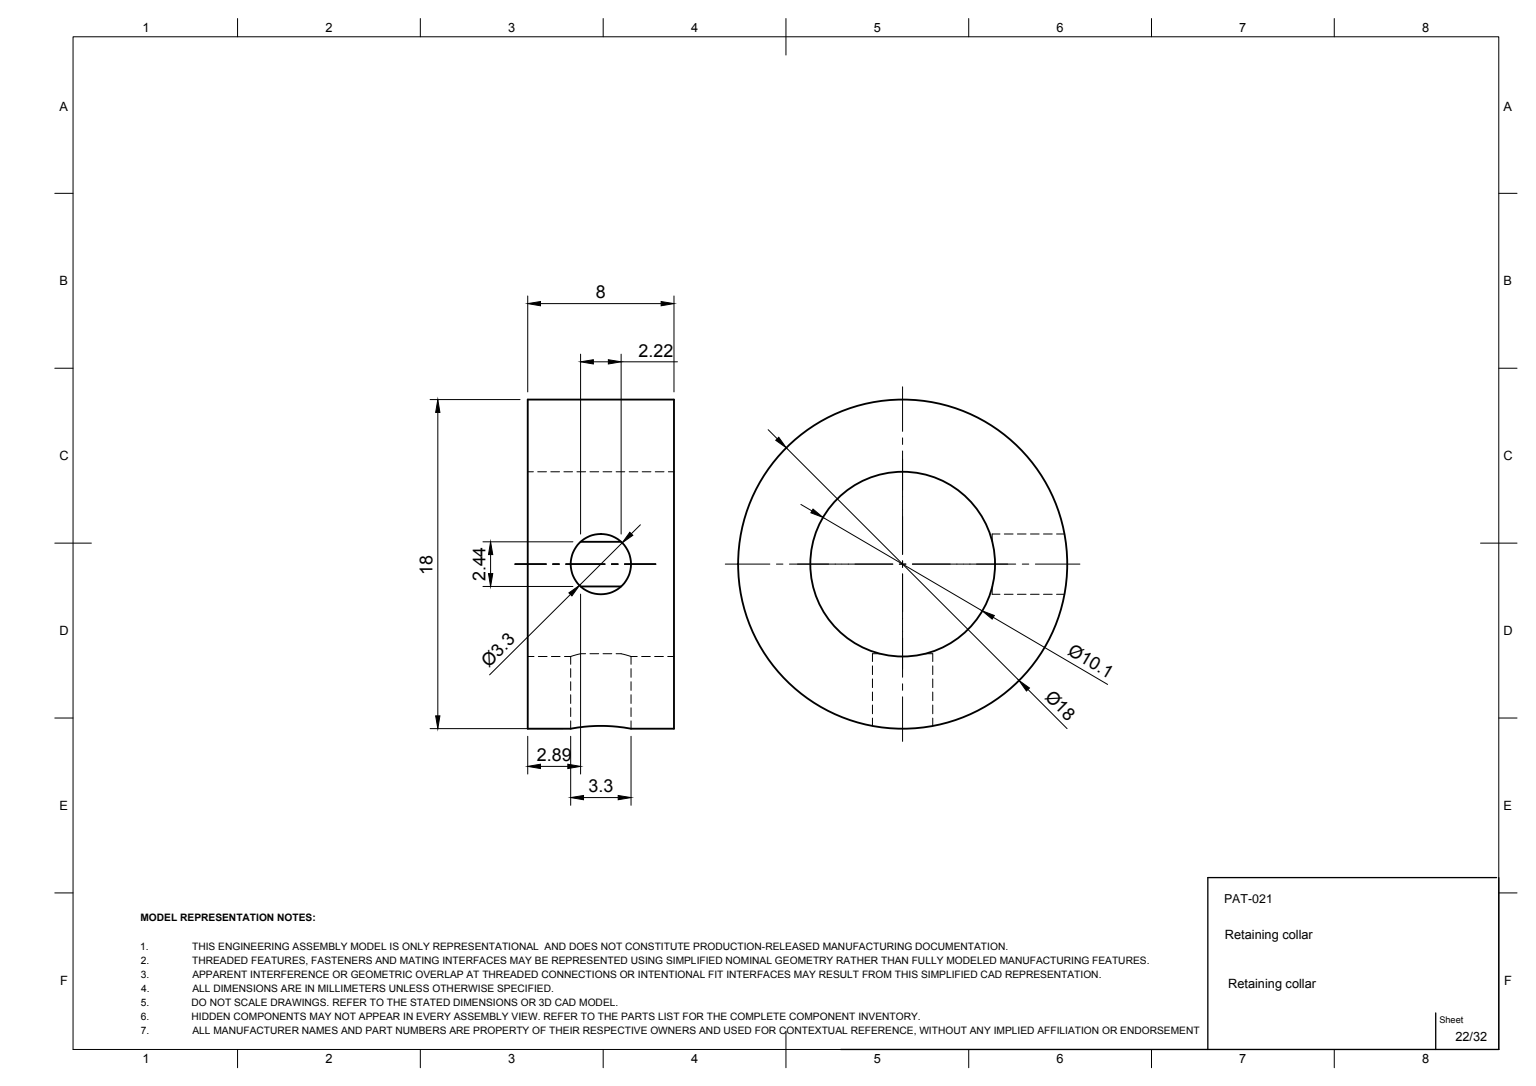
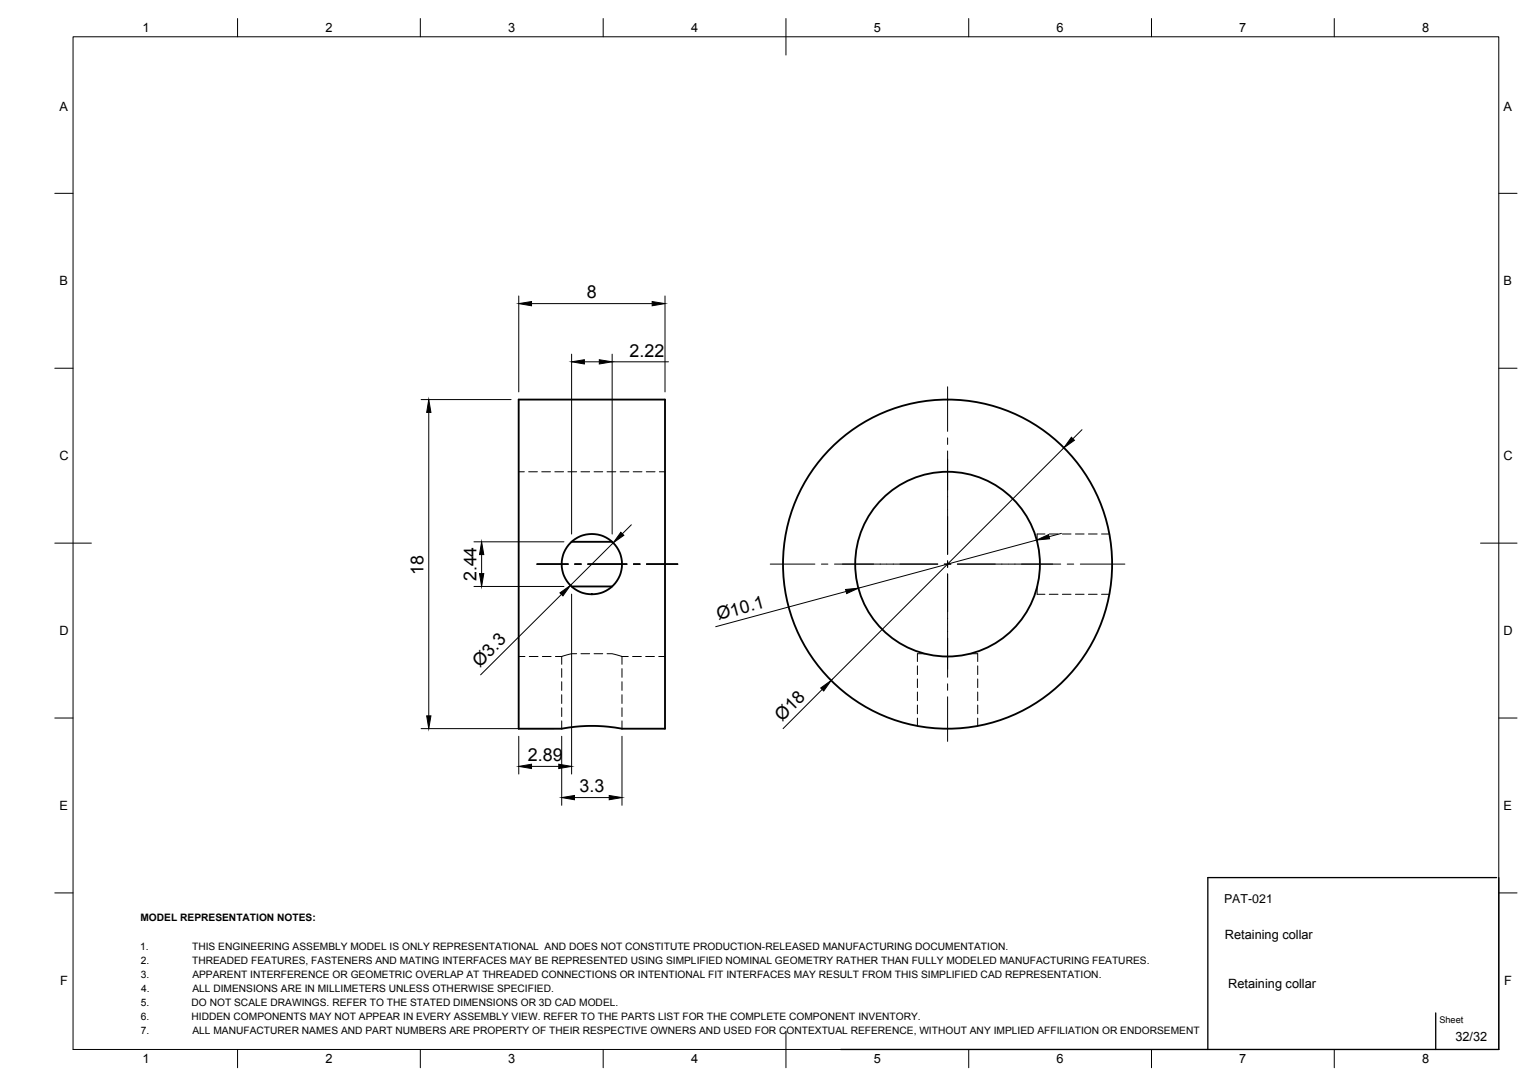
ISO-10303-21;
HEADER;
/* Generated by software containing ST-Developer
 * from STEP Tools, Inc. (www.steptools.com) 
 */

FILE_DESCRIPTION(
/* description */ ('Chain-less indexing wheel (Geneva) drive'),
/* implementation_level */ '2;1');

FILE_NAME(
/* name */ 'Retaining collar.step',
/* time_stamp */ '2026-10-28T03:25:22-07:00',
/* author */ (''),
/* organization */ (''),
/* preprocessor_version */ 'ST-DEVELOPER v20.2',
/* originating_system */ 'Autodesk Translation Framework v15.17.0.0',
/* authorisation */ '');

FILE_SCHEMA (('AUTOMOTIVE_DESIGN { 1 0 10303 214 3 1 1 }'));
ENDSEC;

DATA;
#10=MECHANICAL_DESIGN_GEOMETRIC_PRESENTATION_REPRESENTATION('',(#325),#10957);
#233=B_SPLINE_CURVE_WITH_KNOTS('',3,(#9946,#9947,#9948,#9949,#9950,#9951,
#9952,#9953,#9954,#9955,#9956,#9957,#9958,#9959,#9960,#9961,#9962,#9963,
#9964,#9965,#9966,#9967,#9968,#9969,#9970,#9971,#9972,#9973,#9974,#9975,
#9976,#9977,#9978,#9979),.UNSPECIFIED.,.T.,.F.,(4,2,2,2,2,2,2,2,2,2,2,2,
2,2,2,2,4),(0.,0.0623062782223143,0.124612556444629,0.186916384615149,0.249220212785669,
0.31152404095619,0.37382786912671,0.436134147349024,0.498440425571339,0.560746703793653,
0.623052982015967,0.685356810186488,0.747660638357008,0.809964466527529,
0.872268294698049,0.934574572920363,0.996880851142677),.UNSPECIFIED.);
#234=B_SPLINE_CURVE_WITH_KNOTS('',3,(#9982,#9983,#9984,#9985,#9986,#9987,
#9988,#9989,#9990,#9991,#9992,#9993,#9994,#9995),.UNSPECIFIED.,.F.,.F.,
(4,2,2,2,2,2,4),(0.618551524396292,0.626563103102765,0.689203386094988,
0.751843669087211,0.814483952079434,0.877124235071657,0.88513581377813),
 .UNSPECIFIED.);
#235=B_SPLINE_CURVE_WITH_KNOTS('',3,(#9998,#9999,#10000,#10001,#10002,#10003,
#10004,#10005,#10006,#10007,#10008,#10009,#10010,#10011),.UNSPECIFIED.,
 .F.,.F.,(4,2,2,2,2,2,4),(0.117322411671485,0.125333990377958,0.187974273370181,
0.250614556362404,0.313254839354627,0.37589512234685,0.383906701053323),
 .UNSPECIFIED.);
#236=B_SPLINE_CURVE_WITH_KNOTS('',3,(#10022,#10023,#10024,#10025,#10026,
#10027,#10028,#10029,#10030,#10031),.UNSPECIFIED.,.F.,.F.,(4,2,2,2,4),(0.,
0.0623062782223142,0.124612556444628,0.186916384615149,0.249220212785669),
 .UNSPECIFIED.);
#237=B_SPLINE_CURVE_WITH_KNOTS('',3,(#10033,#10034,#10035,#10036,#10037,
#10038,#10039,#10040,#10041,#10042),.UNSPECIFIED.,.F.,.F.,(4,2,2,2,4),(0.747660638357008,
0.809964466527529,0.872268294698049,0.934574572920363,0.996880851142677),
 .UNSPECIFIED.);
#238=B_SPLINE_CURVE_WITH_KNOTS('',3,(#10043,#10044,#10045,#10046,#10047,
#10048,#10049,#10050,#10051,#10052,#10053,#10054,#10055,#10056,#10057,#10058,
#10059,#10060),.UNSPECIFIED.,.F.,.F.,(4,2,2,2,2,2,2,2,4),(0.249220212785669,
0.31152404095619,0.37382786912671,0.436134147349024,0.498440425571339,0.560746703793653,
0.623052982015967,0.685356810186488,0.747660638357008),.UNSPECIFIED.);
#239=B_SPLINE_CURVE_WITH_KNOTS('',3,(#10064,#10065,#10066,#10067,#10068,
#10069,#10070,#10071),.UNSPECIFIED.,.F.,.F.,(4,2,2,4),(0.618551524396292,
0.626563103102765,0.689203386094988,0.751843669087211),.UNSPECIFIED.);
#240=B_SPLINE_CURVE_WITH_KNOTS('',3,(#10075,#10076,#10077,#10078,#10079,
#10080,#10081,#10082),.UNSPECIFIED.,.F.,.F.,(4,2,2,4),(0.250614556362404,
0.313254839354627,0.37589512234685,0.383906701053323),.UNSPECIFIED.);
#241=B_SPLINE_CURVE_WITH_KNOTS('',3,(#10083,#10084,#10085,#10086,#10087,
#10088,#10089,#10090),.UNSPECIFIED.,.F.,.F.,(4,2,2,4),(0.117322411671484,
0.125333990377958,0.187974273370181,0.250614556362404),.UNSPECIFIED.);
#242=B_SPLINE_CURVE_WITH_KNOTS('',3,(#10091,#10092,#10093,#10094,#10095,
#10096,#10097,#10098),.UNSPECIFIED.,.F.,.F.,(4,2,2,4),(0.751843669087211,
0.814483952079434,0.877124235071657,0.885135813778131),.UNSPECIFIED.);
#267=SHAPE_REPRESENTATION_RELATIONSHIP('SRR','None',#11082,#292);
#292=ADVANCED_BREP_SHAPE_REPRESENTATION('',(#357),#10945);
#325=STYLED_ITEM('',(#11301),#357);
#357=MANIFOLD_SOLID_BREP('Body1',#5722);
#441=FACE_BOUND('',#1265,.T.);
#442=FACE_BOUND('',#1267,.T.);
#443=FACE_BOUND('',#1269,.T.);
#444=FACE_BOUND('',#1271,.T.);
#569=PLANE('',#6451);
#570=PLANE('',#6456);
#571=PLANE('',#6457);
#572=PLANE('',#6461);
#573=PLANE('',#6468);
#574=PLANE('',#6469);
#851=FACE_OUTER_BOUND('',#1258,.T.);
#852=FACE_OUTER_BOUND('',#1259,.T.);
#853=FACE_OUTER_BOUND('',#1260,.T.);
#854=FACE_OUTER_BOUND('',#1261,.T.);
#855=FACE_OUTER_BOUND('',#1262,.T.);
#856=FACE_OUTER_BOUND('',#1263,.T.);
#857=FACE_OUTER_BOUND('',#1264,.T.);
#858=FACE_OUTER_BOUND('',#1266,.T.);
#859=FACE_OUTER_BOUND('',#1268,.T.);
#860=FACE_OUTER_BOUND('',#1270,.T.);
#1258=EDGE_LOOP('',(#4601,#4602,#4603));
#1259=EDGE_LOOP('',(#4604,#4605,#4606,#4607,#4608,#4609,#4610,#4611));
#1260=EDGE_LOOP('',(#4612,#4613));
#1261=EDGE_LOOP('',(#4614,#4615));
#1262=EDGE_LOOP('',(#4616,#4617,#4618,#4619,#4620,#4621,#4622,#4623,#4624,
#4625,#4626));
#1263=EDGE_LOOP('',(#4627,#4628));
#1264=EDGE_LOOP('',(#4629,#4630,#4631,#4632,#4633,#4634,#4635,#4636,#4637,
#4638,#4639,#4640));
#1265=EDGE_LOOP('',(#4641,#4642,#4643,#4644));
#1266=EDGE_LOOP('',(#4645,#4646,#4647,#4648,#4649,#4650,#4651,#4652,#4653));
#1267=EDGE_LOOP('',(#4654));
#1268=EDGE_LOOP('',(#4655));
#1269=EDGE_LOOP('',(#4656));
#1270=EDGE_LOOP('',(#4657));
#1271=EDGE_LOOP('',(#4658));
#1612=LINE('',#9940,#1986);
#1613=LINE('',#9980,#1987);
#1614=LINE('',#10013,#1988);
#1615=LINE('',#10017,#1989);
#1616=LINE('',#10062,#1990);
#1617=LINE('',#10100,#1991);
#1618=LINE('',#10104,#1992);
#1619=LINE('',#10106,#1993);
#1620=LINE('',#10111,#1994);
#1621=LINE('',#10113,#1995);
#1986=VECTOR('',#7822,1.);
#1987=VECTOR('',#7829,0.165);
#1988=VECTOR('',#7834,1.);
#1989=VECTOR('',#7837,1.);
#1990=VECTOR('',#7842,0.165);
#1991=VECTOR('',#7847,1.);
#1992=VECTOR('',#7852,0.505);
#1993=VECTOR('',#7853,0.505);
#1994=VECTOR('',#7860,0.9);
#1995=VECTOR('',#7861,0.9);
#2389=CIRCLE('',#6452,0.165);
#2390=CIRCLE('',#6453,0.165);
#2391=CIRCLE('',#6455,0.165);
#2392=CIRCLE('',#6458,0.165);
#2393=CIRCLE('',#6460,0.165);
#2394=CIRCLE('',#6463,0.505);
#2395=CIRCLE('',#6464,0.505);
#2396=CIRCLE('',#6466,0.9);
#2397=CIRCLE('',#6467,0.9);
#2787=VERTEX_POINT('',#9938);
#2788=VERTEX_POINT('',#9939);
#2789=VERTEX_POINT('',#9941);
#2790=VERTEX_POINT('',#9945);
#2791=VERTEX_POINT('',#9981);
#2792=VERTEX_POINT('',#9996);
#2793=VERTEX_POINT('',#10015);
#2794=VERTEX_POINT('',#10016);
#2795=VERTEX_POINT('',#10020);
#2796=VERTEX_POINT('',#10021);
#2797=VERTEX_POINT('',#10032);
#2798=VERTEX_POINT('',#10061);
#2799=VERTEX_POINT('',#10063);
#2800=VERTEX_POINT('',#10072);
#2801=VERTEX_POINT('',#10074);
#2802=VERTEX_POINT('',#10102);
#2803=VERTEX_POINT('',#10105);
#2804=VERTEX_POINT('',#10109);
#2805=VERTEX_POINT('',#10112);
#3426=EDGE_CURVE('',#2787,#2788,#1612,.T.);
#3427=EDGE_CURVE('',#2789,#2787,#2389,.T.);
#3428=EDGE_CURVE('',#2788,#2789,#2390,.T.);
#3429=EDGE_CURVE('',#2790,#2790,#233,.T.);
#3430=EDGE_CURVE('',#2790,#2789,#1613,.T.);
#3431=EDGE_CURVE('',#2791,#2787,#234,.T.);
#3432=EDGE_CURVE('',#2791,#2792,#2391,.T.);
#3433=EDGE_CURVE('',#2788,#2792,#235,.T.);
#3434=EDGE_CURVE('',#2792,#2791,#1614,.T.);
#3435=EDGE_CURVE('',#2793,#2794,#1615,.T.);
#3436=EDGE_CURVE('',#2794,#2793,#2392,.T.);
#3437=EDGE_CURVE('',#2795,#2796,#236,.T.);
#3438=EDGE_CURVE('',#2797,#2795,#237,.T.);
#3439=EDGE_CURVE('',#2796,#2797,#238,.T.);
#3440=EDGE_CURVE('',#2796,#2798,#1616,.T.);
#3441=EDGE_CURVE('',#2799,#2798,#239,.T.);
#3442=EDGE_CURVE('',#2799,#2800,#2393,.T.);
#3443=EDGE_CURVE('',#2801,#2800,#240,.T.);
#3444=EDGE_CURVE('',#2794,#2801,#241,.T.);
#3445=EDGE_CURVE('',#2798,#2793,#242,.T.);
#3446=EDGE_CURVE('',#2800,#2799,#1617,.T.);
#3447=EDGE_CURVE('',#2802,#2802,#2394,.T.);
#3448=EDGE_CURVE('',#2802,#2798,#1618,.T.);
#3449=EDGE_CURVE('',#2801,#2803,#1619,.T.);
#3450=EDGE_CURVE('',#2803,#2803,#2395,.T.);
#3451=EDGE_CURVE('',#2804,#2804,#2396,.T.);
#3452=EDGE_CURVE('',#2804,#2796,#1620,.T.);
#3453=EDGE_CURVE('',#2797,#2805,#1621,.T.);
#3454=EDGE_CURVE('',#2805,#2805,#2397,.T.);
#4601=ORIENTED_EDGE('',*,*,#3426,.F.);
#4602=ORIENTED_EDGE('',*,*,#3427,.F.);
#4603=ORIENTED_EDGE('',*,*,#3428,.F.);
#4604=ORIENTED_EDGE('',*,*,#3429,.F.);
#4605=ORIENTED_EDGE('',*,*,#3430,.T.);
#4606=ORIENTED_EDGE('',*,*,#3427,.T.);
#4607=ORIENTED_EDGE('',*,*,#3431,.F.);
#4608=ORIENTED_EDGE('',*,*,#3432,.T.);
#4609=ORIENTED_EDGE('',*,*,#3433,.F.);
#4610=ORIENTED_EDGE('',*,*,#3428,.T.);
#4611=ORIENTED_EDGE('',*,*,#3430,.F.);
#4612=ORIENTED_EDGE('',*,*,#3434,.F.);
#4613=ORIENTED_EDGE('',*,*,#3432,.F.);
#4614=ORIENTED_EDGE('',*,*,#3435,.F.);
#4615=ORIENTED_EDGE('',*,*,#3436,.F.);
#4616=ORIENTED_EDGE('',*,*,#3437,.F.);
#4617=ORIENTED_EDGE('',*,*,#3438,.F.);
#4618=ORIENTED_EDGE('',*,*,#3439,.F.);
#4619=ORIENTED_EDGE('',*,*,#3440,.T.);
#4620=ORIENTED_EDGE('',*,*,#3441,.F.);
#4621=ORIENTED_EDGE('',*,*,#3442,.T.);
#4622=ORIENTED_EDGE('',*,*,#3443,.F.);
#4623=ORIENTED_EDGE('',*,*,#3444,.F.);
#4624=ORIENTED_EDGE('',*,*,#3436,.T.);
#4625=ORIENTED_EDGE('',*,*,#3445,.F.);
#4626=ORIENTED_EDGE('',*,*,#3440,.F.);
#4627=ORIENTED_EDGE('',*,*,#3446,.F.);
#4628=ORIENTED_EDGE('',*,*,#3442,.F.);
#4629=ORIENTED_EDGE('',*,*,#3447,.F.);
#4630=ORIENTED_EDGE('',*,*,#3448,.T.);
#4631=ORIENTED_EDGE('',*,*,#3445,.T.);
#4632=ORIENTED_EDGE('',*,*,#3435,.T.);
#4633=ORIENTED_EDGE('',*,*,#3444,.T.);
#4634=ORIENTED_EDGE('',*,*,#3449,.T.);
#4635=ORIENTED_EDGE('',*,*,#3450,.T.);
#4636=ORIENTED_EDGE('',*,*,#3449,.F.);
#4637=ORIENTED_EDGE('',*,*,#3443,.T.);
#4638=ORIENTED_EDGE('',*,*,#3446,.T.);
#4639=ORIENTED_EDGE('',*,*,#3441,.T.);
#4640=ORIENTED_EDGE('',*,*,#3448,.F.);
#4641=ORIENTED_EDGE('',*,*,#3433,.T.);
#4642=ORIENTED_EDGE('',*,*,#3434,.T.);
#4643=ORIENTED_EDGE('',*,*,#3431,.T.);
#4644=ORIENTED_EDGE('',*,*,#3426,.T.);
#4645=ORIENTED_EDGE('',*,*,#3451,.F.);
#4646=ORIENTED_EDGE('',*,*,#3452,.T.);
#4647=ORIENTED_EDGE('',*,*,#3439,.T.);
#4648=ORIENTED_EDGE('',*,*,#3453,.T.);
#4649=ORIENTED_EDGE('',*,*,#3454,.T.);
#4650=ORIENTED_EDGE('',*,*,#3453,.F.);
#4651=ORIENTED_EDGE('',*,*,#3438,.T.);
#4652=ORIENTED_EDGE('',*,*,#3437,.T.);
#4653=ORIENTED_EDGE('',*,*,#3452,.F.);
#4654=ORIENTED_EDGE('',*,*,#3429,.T.);
#4655=ORIENTED_EDGE('',*,*,#3451,.T.);
#4656=ORIENTED_EDGE('',*,*,#3447,.T.);
#4657=ORIENTED_EDGE('',*,*,#3454,.F.);
#4658=ORIENTED_EDGE('',*,*,#3450,.F.);
#5319=CYLINDRICAL_SURFACE('',#6454,0.165);
#5320=CYLINDRICAL_SURFACE('',#6459,0.165);
#5321=CYLINDRICAL_SURFACE('',#6462,0.505);
#5322=CYLINDRICAL_SURFACE('',#6465,0.9);
#5565=ADVANCED_FACE('',(#851),#569,.F.);
#5566=ADVANCED_FACE('',(#852),#5319,.F.);
#5567=ADVANCED_FACE('',(#853),#570,.F.);
#5568=ADVANCED_FACE('',(#854),#571,.F.);
#5569=ADVANCED_FACE('',(#855),#5320,.F.);
#5570=ADVANCED_FACE('',(#856),#572,.F.);
#5571=ADVANCED_FACE('',(#857,#441),#5321,.F.);
#5572=ADVANCED_FACE('',(#858,#442),#5322,.T.);
#5573=ADVANCED_FACE('',(#859,#443),#573,.T.);
#5574=ADVANCED_FACE('',(#860,#444),#574,.F.);
#5722=CLOSED_SHELL('',(#5565,#5566,#5567,#5568,#5569,#5570,#5571,#5572,
#5573,#5574));
#6450=AXIS2_PLACEMENT_3D('',#9936,#7818,#7819);
#6451=AXIS2_PLACEMENT_3D('',#9937,#7820,#7821);
#6452=AXIS2_PLACEMENT_3D('',#9942,#7823,#7824);
#6453=AXIS2_PLACEMENT_3D('',#9943,#7825,#7826);
#6454=AXIS2_PLACEMENT_3D('',#9944,#7827,#7828);
#6455=AXIS2_PLACEMENT_3D('',#9997,#7830,#7831);
#6456=AXIS2_PLACEMENT_3D('',#10012,#7832,#7833);
#6457=AXIS2_PLACEMENT_3D('',#10014,#7835,#7836);
#6458=AXIS2_PLACEMENT_3D('',#10018,#7838,#7839);
#6459=AXIS2_PLACEMENT_3D('',#10019,#7840,#7841);
#6460=AXIS2_PLACEMENT_3D('',#10073,#7843,#7844);
#6461=AXIS2_PLACEMENT_3D('',#10099,#7845,#7846);
#6462=AXIS2_PLACEMENT_3D('',#10101,#7848,#7849);
#6463=AXIS2_PLACEMENT_3D('',#10103,#7850,#7851);
#6464=AXIS2_PLACEMENT_3D('',#10107,#7854,#7855);
#6465=AXIS2_PLACEMENT_3D('',#10108,#7856,#7857);
#6466=AXIS2_PLACEMENT_3D('',#10110,#7858,#7859);
#6467=AXIS2_PLACEMENT_3D('',#10114,#7862,#7863);
#6468=AXIS2_PLACEMENT_3D('',#10115,#7864,#7865);
#6469=AXIS2_PLACEMENT_3D('',#10116,#7866,#7867);
#7818=DIRECTION('axis',(0.,0.,1.));
#7819=DIRECTION('refdir',(1.,0.,0.));
#7820=DIRECTION('center_axis',(0.,1.,0.));
#7821=DIRECTION('ref_axis',(1.,0.,0.));
#7822=DIRECTION('',(0.,0.,-1.));
#7823=DIRECTION('center_axis',(0.,1.,0.));
#7824=DIRECTION('ref_axis',(1.,0.,0.));
#7825=DIRECTION('center_axis',(0.,1.,0.));
#7826=DIRECTION('ref_axis',(1.,0.,0.));
#7827=DIRECTION('center_axis',(0.,1.,0.));
#7828=DIRECTION('ref_axis',(1.,0.,0.));
#7829=DIRECTION('',(0.,1.,0.));
#7830=DIRECTION('center_axis',(0.,1.,0.));
#7831=DIRECTION('ref_axis',(1.,0.,0.));
#7832=DIRECTION('center_axis',(0.,1.,0.));
#7833=DIRECTION('ref_axis',(1.,0.,0.));
#7834=DIRECTION('',(0.,0.,1.));
#7835=DIRECTION('center_axis',(1.,0.,0.));
#7836=DIRECTION('ref_axis',(0.,0.,-1.));
#7837=DIRECTION('',(0.,0.,-1.));
#7838=DIRECTION('center_axis',(1.,0.,0.));
#7839=DIRECTION('ref_axis',(0.,0.,-1.));
#7840=DIRECTION('center_axis',(1.,0.,0.));
#7841=DIRECTION('ref_axis',(0.,0.,-1.));
#7842=DIRECTION('',(1.,0.,0.));
#7843=DIRECTION('center_axis',(1.,0.,0.));
#7844=DIRECTION('ref_axis',(0.,0.,-1.));
#7845=DIRECTION('center_axis',(1.,0.,0.));
#7846=DIRECTION('ref_axis',(0.,0.,-1.));
#7847=DIRECTION('',(0.,0.,1.));
#7848=DIRECTION('center_axis',(0.,0.,1.));
#7849=DIRECTION('ref_axis',(1.,0.,0.));
#7850=DIRECTION('center_axis',(0.,0.,-1.));
#7851=DIRECTION('ref_axis',(1.,0.,0.));
#7852=DIRECTION('',(0.,0.,-1.));
#7853=DIRECTION('',(0.,0.,-1.));
#7854=DIRECTION('center_axis',(0.,0.,-1.));
#7855=DIRECTION('ref_axis',(1.,0.,0.));
#7856=DIRECTION('center_axis',(0.,0.,1.));
#7857=DIRECTION('ref_axis',(1.,0.,0.));
#7858=DIRECTION('center_axis',(0.,0.,1.));
#7859=DIRECTION('ref_axis',(1.,0.,0.));
#7860=DIRECTION('',(0.,0.,-1.));
#7861=DIRECTION('',(0.,0.,-1.));
#7862=DIRECTION('center_axis',(0.,0.,1.));
#7863=DIRECTION('ref_axis',(1.,0.,0.));
#7864=DIRECTION('center_axis',(0.,0.,1.));
#7865=DIRECTION('ref_axis',(1.,0.,0.));
#7866=DIRECTION('center_axis',(0.,0.,1.));
#7867=DIRECTION('ref_axis',(1.,0.,0.));
#9936=CARTESIAN_POINT('',(0.,0.,0.));
#9937=CARTESIAN_POINT('Origin',(0.,-0.49,1.4));
#9938=CARTESIAN_POINT('',(-0.122167917228706,-0.49,1.51090536506409));
#9939=CARTESIAN_POINT('',(-0.122167917228706,-0.49,1.28909463493591));
#9940=CARTESIAN_POINT('',(-0.122167917228706,-0.49,1.));
#9941=CARTESIAN_POINT('',(-0.165,-0.49,1.4));
#9942=CARTESIAN_POINT('Origin',(0.,-0.49,1.4));
#9943=CARTESIAN_POINT('Origin',(0.,-0.49,1.4));
#9944=CARTESIAN_POINT('Origin',(0.,-1.,1.4));
#9945=CARTESIAN_POINT('',(-0.165,-0.884745726183518,1.4));
#9946=CARTESIAN_POINT('Ctrl Pts',(-0.165,-0.884745726183518,1.4));
#9947=CARTESIAN_POINT('Ctrl Pts',(-0.165,-0.884745726183518,1.42076875940744));
#9948=CARTESIAN_POINT('Ctrl Pts',(-0.160839719007584,-0.885552759505264,
1.44288889507334));
#9949=CARTESIAN_POINT('Ctrl Pts',(-0.14398647021669,-0.888448648150043,
1.48352706263377));
#9950=CARTESIAN_POINT('Ctrl Pts',(-0.131295993814186,-0.890493604851638,
1.50204924397737));
#9951=CARTESIAN_POINT('Ctrl Pts',(-0.102049819008125,-0.89431723432394,
1.53129541878344));
#9952=CARTESIAN_POINT('Ctrl Pts',(-0.0835273920906823,-0.896347088899543,
1.54398634598358));
#9953=CARTESIAN_POINT('Ctrl Pts',(-0.0428883760934128,-0.899208271860583,
1.56083992183864));
#9954=CARTESIAN_POINT('Ctrl Pts',(-0.0207679427235068,-0.9,1.565));
#9955=CARTESIAN_POINT('Ctrl Pts',(0.0207679427235068,-0.9,1.565));
#9956=CARTESIAN_POINT('Ctrl Pts',(0.0428883760934127,-0.899208271860583,
1.56083992183864));
#9957=CARTESIAN_POINT('Ctrl Pts',(0.0835273920906823,-0.896347088899543,
1.54398634598358));
#9958=CARTESIAN_POINT('Ctrl Pts',(0.102049819008125,-0.89431723432394,1.53129541878344));
#9959=CARTESIAN_POINT('Ctrl Pts',(0.131295993814186,-0.890493604851638,
1.50204924397737));
#9960=CARTESIAN_POINT('Ctrl Pts',(0.14398647021669,-0.888448648150043,1.48352706263377));
#9961=CARTESIAN_POINT('Ctrl Pts',(0.160839719007584,-0.885552759505264,
1.44288889507334));
#9962=CARTESIAN_POINT('Ctrl Pts',(0.165,-0.884745726183518,1.42076875940744));
#9963=CARTESIAN_POINT('Ctrl Pts',(0.165,-0.884745726183518,1.37923124059256));
#9964=CARTESIAN_POINT('Ctrl Pts',(0.160839719007584,-0.885552759505264,
1.35711110492666));
#9965=CARTESIAN_POINT('Ctrl Pts',(0.14398647021669,-0.888448648150043,1.31647293736623));
#9966=CARTESIAN_POINT('Ctrl Pts',(0.131295993814186,-0.890493604851638,
1.29795075602263));
#9967=CARTESIAN_POINT('Ctrl Pts',(0.102049819008125,-0.89431723432394,1.26870458121656));
#9968=CARTESIAN_POINT('Ctrl Pts',(0.0835273920906823,-0.896347088899543,
1.25601365401642));
#9969=CARTESIAN_POINT('Ctrl Pts',(0.0428883760934127,-0.899208271860583,
1.23916007816136));
#9970=CARTESIAN_POINT('Ctrl Pts',(0.0207679427235068,-0.9,1.235));
#9971=CARTESIAN_POINT('Ctrl Pts',(-0.0207679427235067,-0.9,1.235));
#9972=CARTESIAN_POINT('Ctrl Pts',(-0.0428883760934127,-0.899208271860583,
1.23916007816136));
#9973=CARTESIAN_POINT('Ctrl Pts',(-0.0835273920906822,-0.896347088899543,
1.25601365401642));
#9974=CARTESIAN_POINT('Ctrl Pts',(-0.102049819008125,-0.89431723432394,
1.26870458121656));
#9975=CARTESIAN_POINT('Ctrl Pts',(-0.131295993814186,-0.890493604851638,
1.29795075602263));
#9976=CARTESIAN_POINT('Ctrl Pts',(-0.14398647021669,-0.888448648150043,
1.31647293736623));
#9977=CARTESIAN_POINT('Ctrl Pts',(-0.160839719007584,-0.885552759505264,
1.35711110492666));
#9978=CARTESIAN_POINT('Ctrl Pts',(-0.165,-0.884745726183518,1.37923124059256));
#9979=CARTESIAN_POINT('Ctrl Pts',(-0.165,-0.884745726183518,1.4));
#9980=CARTESIAN_POINT('',(-0.165,-1.,1.4));
#9981=CARTESIAN_POINT('',(0.122167917228706,-0.49,1.51090536506409));
#9982=CARTESIAN_POINT('Ctrl Pts',(0.122167917228706,-0.49,1.51090536506409));
#9983=CARTESIAN_POINT('Ctrl Pts',(0.120368913626296,-0.490448531679987,
1.51288705930464));
#9984=CARTESIAN_POINT('Ctrl Pts',(0.118534896565231,-0.490895245371684,
1.51481034122633));
#9985=CARTESIAN_POINT('Ctrl Pts',(0.102111993019358,-0.494795015531646,
1.5312332447722));
#9986=CARTESIAN_POINT('Ctrl Pts',(0.0836597150224318,-0.498442514607594,
1.54390845611142));
#9987=CARTESIAN_POINT('Ctrl Pts',(0.0430495960471595,-0.50357781976106,
1.56079590960766));
#9988=CARTESIAN_POINT('Ctrl Pts',(0.020880094330741,-0.505,1.565));
#9989=CARTESIAN_POINT('Ctrl Pts',(-0.020880094330741,-0.505,1.565));
#9990=CARTESIAN_POINT('Ctrl Pts',(-0.0430495960471594,-0.50357781976106,
1.56079590960766));
#9991=CARTESIAN_POINT('Ctrl Pts',(-0.0836597150224317,-0.498442514607594,
1.54390845611142));
#9992=CARTESIAN_POINT('Ctrl Pts',(-0.102111993019358,-0.494795015531646,
1.5312332447722));
#9993=CARTESIAN_POINT('Ctrl Pts',(-0.118534896565231,-0.490895245371684,
1.51481034122633));
#9994=CARTESIAN_POINT('Ctrl Pts',(-0.120368913626296,-0.490448531679987,
1.51288705930464));
#9995=CARTESIAN_POINT('Ctrl Pts',(-0.122167917228706,-0.49,1.51090536506409));
#9996=CARTESIAN_POINT('',(0.122167917228706,-0.49,1.28909463493591));
#9997=CARTESIAN_POINT('Origin',(0.,-0.49,1.4));
#9998=CARTESIAN_POINT('Ctrl Pts',(-0.122167917228706,-0.49,1.28909463493591));
#9999=CARTESIAN_POINT('Ctrl Pts',(-0.120368913626296,-0.490448531679987,
1.28711294069536));
#10000=CARTESIAN_POINT('Ctrl Pts',(-0.118534896565231,-0.490895245371684,
1.28518965877367));
#10001=CARTESIAN_POINT('Ctrl Pts',(-0.102111993019358,-0.494795015531646,
1.2687667552278));
#10002=CARTESIAN_POINT('Ctrl Pts',(-0.0836597150224318,-0.498442514607594,
1.25609154388858));
#10003=CARTESIAN_POINT('Ctrl Pts',(-0.0430495960471595,-0.50357781976106,
1.23920409039234));
#10004=CARTESIAN_POINT('Ctrl Pts',(-0.020880094330741,-0.505,1.235));
#10005=CARTESIAN_POINT('Ctrl Pts',(0.020880094330741,-0.505,1.235));
#10006=CARTESIAN_POINT('Ctrl Pts',(0.0430495960471595,-0.50357781976106,
1.23920409039234));
#10007=CARTESIAN_POINT('Ctrl Pts',(0.0836597150224318,-0.498442514607594,
1.25609154388858));
#10008=CARTESIAN_POINT('Ctrl Pts',(0.102111993019358,-0.494795015531646,
1.2687667552278));
#10009=CARTESIAN_POINT('Ctrl Pts',(0.118534896565231,-0.490895245371684,
1.28518965877367));
#10010=CARTESIAN_POINT('Ctrl Pts',(0.120368913626296,-0.490448531679987,
1.28711294069536));
#10011=CARTESIAN_POINT('Ctrl Pts',(0.122167917228706,-0.49,1.28909463493591));
#10012=CARTESIAN_POINT('Origin',(0.,-0.49,1.4));
#10013=CARTESIAN_POINT('',(0.122167917228706,-0.49,1.));
#10014=CARTESIAN_POINT('Origin',(-0.49,0.,1.4));
#10015=CARTESIAN_POINT('',(-0.49,0.122167917228706,1.51090536506409));
#10016=CARTESIAN_POINT('',(-0.49,0.122167917228706,1.28909463493591));
#10017=CARTESIAN_POINT('',(-0.49,0.122167917228706,1.));
#10018=CARTESIAN_POINT('Origin',(-0.49,0.,1.4));
#10019=CARTESIAN_POINT('Origin',(-1.,0.,1.4));
#10020=CARTESIAN_POINT('',(-0.884745726183518,0.165,1.4));
#10021=CARTESIAN_POINT('',(-0.9,-2.02066721859313E-17,1.565));
#10022=CARTESIAN_POINT('Ctrl Pts',(-0.884745726183518,0.165,1.4));
#10023=CARTESIAN_POINT('Ctrl Pts',(-0.884745726183518,0.165,1.42076875940744));
#10024=CARTESIAN_POINT('Ctrl Pts',(-0.885552759505264,0.160839719007584,
1.44288889507334));
#10025=CARTESIAN_POINT('Ctrl Pts',(-0.888448648150043,0.14398647021669,
1.48352706263377));
#10026=CARTESIAN_POINT('Ctrl Pts',(-0.890493604851638,0.131295993814186,
1.50204924397737));
#10027=CARTESIAN_POINT('Ctrl Pts',(-0.89431723432394,0.102049819008125,
1.53129541878344));
#10028=CARTESIAN_POINT('Ctrl Pts',(-0.896347088899543,0.0835273920906824,
1.54398634598358));
#10029=CARTESIAN_POINT('Ctrl Pts',(-0.899208271860583,0.0428883760934128,
1.56083992183864));
#10030=CARTESIAN_POINT('Ctrl Pts',(-0.9,0.0207679427235068,1.565));
#10031=CARTESIAN_POINT('Ctrl Pts',(-0.9,2.77555756156289E-17,1.565));
#10032=CARTESIAN_POINT('',(-0.9,-8.63341285292134E-17,1.235));
#10033=CARTESIAN_POINT('Ctrl Pts',(-0.9,-6.24500451351651E-17,1.235));
#10034=CARTESIAN_POINT('Ctrl Pts',(-0.9,0.0207679427235068,1.235));
#10035=CARTESIAN_POINT('Ctrl Pts',(-0.899208271860583,0.0428883760934128,
1.23916007816136));
#10036=CARTESIAN_POINT('Ctrl Pts',(-0.896347088899543,0.0835273920906824,
1.25601365401642));
#10037=CARTESIAN_POINT('Ctrl Pts',(-0.89431723432394,0.102049819008125,
1.26870458121656));
#10038=CARTESIAN_POINT('Ctrl Pts',(-0.890493604851638,0.131295993814186,
1.29795075602263));
#10039=CARTESIAN_POINT('Ctrl Pts',(-0.888448648150043,0.143986470216691,
1.31647293736623));
#10040=CARTESIAN_POINT('Ctrl Pts',(-0.885552759505264,0.160839719007584,
1.35711110492666));
#10041=CARTESIAN_POINT('Ctrl Pts',(-0.884745726183518,0.165,1.37923124059256));
#10042=CARTESIAN_POINT('Ctrl Pts',(-0.884745726183518,0.165,1.4));
#10043=CARTESIAN_POINT('Ctrl Pts',(-0.9,4.16333634234434E-17,1.565));
#10044=CARTESIAN_POINT('Ctrl Pts',(-0.9,-0.0207679427235068,1.565));
#10045=CARTESIAN_POINT('Ctrl Pts',(-0.899208271860583,-0.0428883760934127,
1.56083992183864));
#10046=CARTESIAN_POINT('Ctrl Pts',(-0.896347088899543,-0.0835273920906824,
1.54398634598358));
#10047=CARTESIAN_POINT('Ctrl Pts',(-0.89431723432394,-0.102049819008125,
1.53129541878344));
#10048=CARTESIAN_POINT('Ctrl Pts',(-0.890493604851638,-0.131295993814186,
1.50204924397737));
#10049=CARTESIAN_POINT('Ctrl Pts',(-0.888448648150043,-0.143986470216691,
1.48352706263377));
#10050=CARTESIAN_POINT('Ctrl Pts',(-0.885552759505264,-0.160839719007584,
1.44288889507334));
#10051=CARTESIAN_POINT('Ctrl Pts',(-0.884745726183518,-0.165,1.42076875940744));
#10052=CARTESIAN_POINT('Ctrl Pts',(-0.884745726183518,-0.165,1.37923124059256));
#10053=CARTESIAN_POINT('Ctrl Pts',(-0.885552759505264,-0.160839719007584,
1.35711110492666));
#10054=CARTESIAN_POINT('Ctrl Pts',(-0.888448648150043,-0.14398647021669,
1.31647293736623));
#10055=CARTESIAN_POINT('Ctrl Pts',(-0.890493604851638,-0.131295993814186,
1.29795075602263));
#10056=CARTESIAN_POINT('Ctrl Pts',(-0.89431723432394,-0.102049819008125,
1.26870458121656));
#10057=CARTESIAN_POINT('Ctrl Pts',(-0.896347088899543,-0.0835273920906825,
1.25601365401642));
#10058=CARTESIAN_POINT('Ctrl Pts',(-0.899208271860583,-0.0428883760934129,
1.23916007816136));
#10059=CARTESIAN_POINT('Ctrl Pts',(-0.9,-0.0207679427235069,1.235));
#10060=CARTESIAN_POINT('Ctrl Pts',(-0.9,-4.85722573273506E-17,1.235));
#10061=CARTESIAN_POINT('',(-0.505,-2.74505708527337E-17,1.565));
#10062=CARTESIAN_POINT('',(-1.,-2.02066721859313E-17,1.565));
#10063=CARTESIAN_POINT('',(-0.49,-0.122167917228706,1.51090536506409));
#10064=CARTESIAN_POINT('Ctrl Pts',(-0.49,-0.122167917228706,1.51090536506409));
#10065=CARTESIAN_POINT('Ctrl Pts',(-0.490448531679987,-0.120368913626296,
1.51288705930464));
#10066=CARTESIAN_POINT('Ctrl Pts',(-0.490895245371684,-0.118534896565231,
1.51481034122633));
#10067=CARTESIAN_POINT('Ctrl Pts',(-0.494795015531646,-0.102111993019358,
1.5312332447722));
#10068=CARTESIAN_POINT('Ctrl Pts',(-0.498442514607594,-0.0836597150224318,
1.54390845611142));
#10069=CARTESIAN_POINT('Ctrl Pts',(-0.50357781976106,-0.0430495960471595,
1.56079590960766));
#10070=CARTESIAN_POINT('Ctrl Pts',(-0.505,-0.020880094330741,1.565));
#10071=CARTESIAN_POINT('Ctrl Pts',(-0.505,0.,1.565));
#10072=CARTESIAN_POINT('',(-0.49,-0.122167917228706,1.28909463493591));
#10073=CARTESIAN_POINT('Origin',(-0.49,0.,1.4));
#10074=CARTESIAN_POINT('',(-0.505,-2.05139908226098E-17,1.235));
#10075=CARTESIAN_POINT('Ctrl Pts',(-0.505,2.77555756156289E-17,1.235));
#10076=CARTESIAN_POINT('Ctrl Pts',(-0.505,-0.020880094330741,1.235));
#10077=CARTESIAN_POINT('Ctrl Pts',(-0.50357781976106,-0.0430495960471594,
1.23920409039234));
#10078=CARTESIAN_POINT('Ctrl Pts',(-0.498442514607595,-0.0836597150224317,
1.25609154388858));
#10079=CARTESIAN_POINT('Ctrl Pts',(-0.494795015531646,-0.102111993019358,
1.2687667552278));
#10080=CARTESIAN_POINT('Ctrl Pts',(-0.490895245371684,-0.118534896565231,
1.28518965877367));
#10081=CARTESIAN_POINT('Ctrl Pts',(-0.490448531679987,-0.120368913626296,
1.28711294069536));
#10082=CARTESIAN_POINT('Ctrl Pts',(-0.49,-0.122167917228706,1.28909463493591));
#10083=CARTESIAN_POINT('Ctrl Pts',(-0.49,0.122167917228706,1.28909463493591));
#10084=CARTESIAN_POINT('Ctrl Pts',(-0.490448531679987,0.120368913626296,
1.28711294069536));
#10085=CARTESIAN_POINT('Ctrl Pts',(-0.490895245371684,0.118534896565231,
1.28518965877367));
#10086=CARTESIAN_POINT('Ctrl Pts',(-0.494795015531646,0.102111993019358,
1.2687667552278));
#10087=CARTESIAN_POINT('Ctrl Pts',(-0.498442514607594,0.0836597150224318,
1.25609154388858));
#10088=CARTESIAN_POINT('Ctrl Pts',(-0.50357781976106,0.0430495960471595,
1.23920409039234));
#10089=CARTESIAN_POINT('Ctrl Pts',(-0.505,0.020880094330741,1.235));
#10090=CARTESIAN_POINT('Ctrl Pts',(-0.505,-6.93889390390723E-18,1.235));
#10091=CARTESIAN_POINT('Ctrl Pts',(-0.505,-2.77555756156289E-17,1.565));
#10092=CARTESIAN_POINT('Ctrl Pts',(-0.505,0.020880094330741,1.565));
#10093=CARTESIAN_POINT('Ctrl Pts',(-0.50357781976106,0.0430495960471595,
1.56079590960766));
#10094=CARTESIAN_POINT('Ctrl Pts',(-0.498442514607594,0.0836597150224318,
1.54390845611142));
#10095=CARTESIAN_POINT('Ctrl Pts',(-0.494795015531646,0.102111993019358,
1.5312332447722));
#10096=CARTESIAN_POINT('Ctrl Pts',(-0.490895245371684,0.118534896565231,
1.51481034122633));
#10097=CARTESIAN_POINT('Ctrl Pts',(-0.490448531679987,0.120368913626296,
1.51288705930464));
#10098=CARTESIAN_POINT('Ctrl Pts',(-0.49,0.122167917228706,1.51090536506409));
#10099=CARTESIAN_POINT('Origin',(-0.49,0.,1.4));
#10100=CARTESIAN_POINT('',(-0.49,-0.122167917228706,1.));
#10101=CARTESIAN_POINT('Origin',(0.,0.,1.));
#10102=CARTESIAN_POINT('',(-0.505,-6.18446633569413E-17,1.8));
#10103=CARTESIAN_POINT('Origin',(0.,0.,1.8));
#10104=CARTESIAN_POINT('',(-0.505,-6.18446633569413E-17,1.));
#10105=CARTESIAN_POINT('',(-0.505,-6.18446633569413E-17,1.));
#10106=CARTESIAN_POINT('',(-0.505,-6.18446633569413E-17,1.));
#10107=CARTESIAN_POINT('Origin',(0.,0.,1.));
#10108=CARTESIAN_POINT('Origin',(0.,0.,1.));
#10109=CARTESIAN_POINT('',(-0.9,-1.10218211923262E-16,1.8));
#10110=CARTESIAN_POINT('Origin',(0.,0.,1.8));
#10111=CARTESIAN_POINT('',(-0.9,-1.10218211923262E-16,1.));
#10112=CARTESIAN_POINT('',(-0.9,-1.10218211923262E-16,1.));
#10113=CARTESIAN_POINT('',(-0.9,-1.10218211923262E-16,1.));
#10114=CARTESIAN_POINT('Origin',(0.,0.,1.));
#10115=CARTESIAN_POINT('Origin',(0.,0.,1.8));
#10116=CARTESIAN_POINT('Origin',(0.,0.,1.));
#10914=UNCERTAINTY_MEASURE_WITH_UNIT(LENGTH_MEASURE(0.001),#10958,
'DISTANCE_ACCURACY_VALUE',
'Maximum model space distance between geometric entities at asserted c
onnectivities');
#10926=UNCERTAINTY_MEASURE_WITH_UNIT(LENGTH_MEASURE(0.001),#10958,
'DISTANCE_ACCURACY_VALUE',
'Maximum model space distance between geometric entities at asserted c
onnectivities');
#10945=(
GEOMETRIC_REPRESENTATION_CONTEXT(3)
GLOBAL_UNCERTAINTY_ASSIGNED_CONTEXT((#10914))
GLOBAL_UNIT_ASSIGNED_CONTEXT((#10958,#10960,#10961))
REPRESENTATION_CONTEXT('','3D')
);
#10957=(
GEOMETRIC_REPRESENTATION_CONTEXT(3)
GLOBAL_UNCERTAINTY_ASSIGNED_CONTEXT((#10926))
GLOBAL_UNIT_ASSIGNED_CONTEXT((#10958,#10960,#10961))
REPRESENTATION_CONTEXT('','3D')
);
#10958=(
LENGTH_UNIT()
NAMED_UNIT(*)
SI_UNIT(.CENTI.,.METRE.)
);
#10960=(
NAMED_UNIT(*)
PLANE_ANGLE_UNIT()
SI_UNIT($,.RADIAN.)
);
#10961=(
NAMED_UNIT(*)
SI_UNIT($,.STERADIAN.)
SOLID_ANGLE_UNIT()
);
#10980=SHAPE_DEFINITION_REPRESENTATION(#11015,#11082);
#11015=PRODUCT_DEFINITION_SHAPE('',$,#11113);
#11082=SHAPE_REPRESENTATION('',(#6450),#10945);
#11094=PRODUCT_DEFINITION_CONTEXT('part definition',#11186,'design');
#11113=PRODUCT_DEFINITION('Retaining collar','Retaining collar',#11143,
#11094);
#11143=PRODUCT_DEFINITION_FORMATION('',$,#11206);
#11186=APPLICATION_CONTEXT(
'Core Data for Automotive Mechanical Design Process');
#11187=PRODUCT_CONTEXT('part definition',#11186,'mechanical');
#11206=PRODUCT('Retaining collar','Retaining collar','Retaining collar',
(#11187));
#11295=COLOUR_RGB('Off White',0.89,0.88,0.83);
#11296=FILL_AREA_STYLE_COLOUR('',#11295);
#11297=FILL_AREA_STYLE('',(#11296));
#11298=SURFACE_STYLE_FILL_AREA(#11297);
#11299=SURFACE_SIDE_STYLE('',(#11298));
#11300=SURFACE_STYLE_USAGE(.BOTH.,#11299);
#11301=PRESENTATION_STYLE_ASSIGNMENT((#11300));
ENDSEC;
END-ISO-10303-21;
